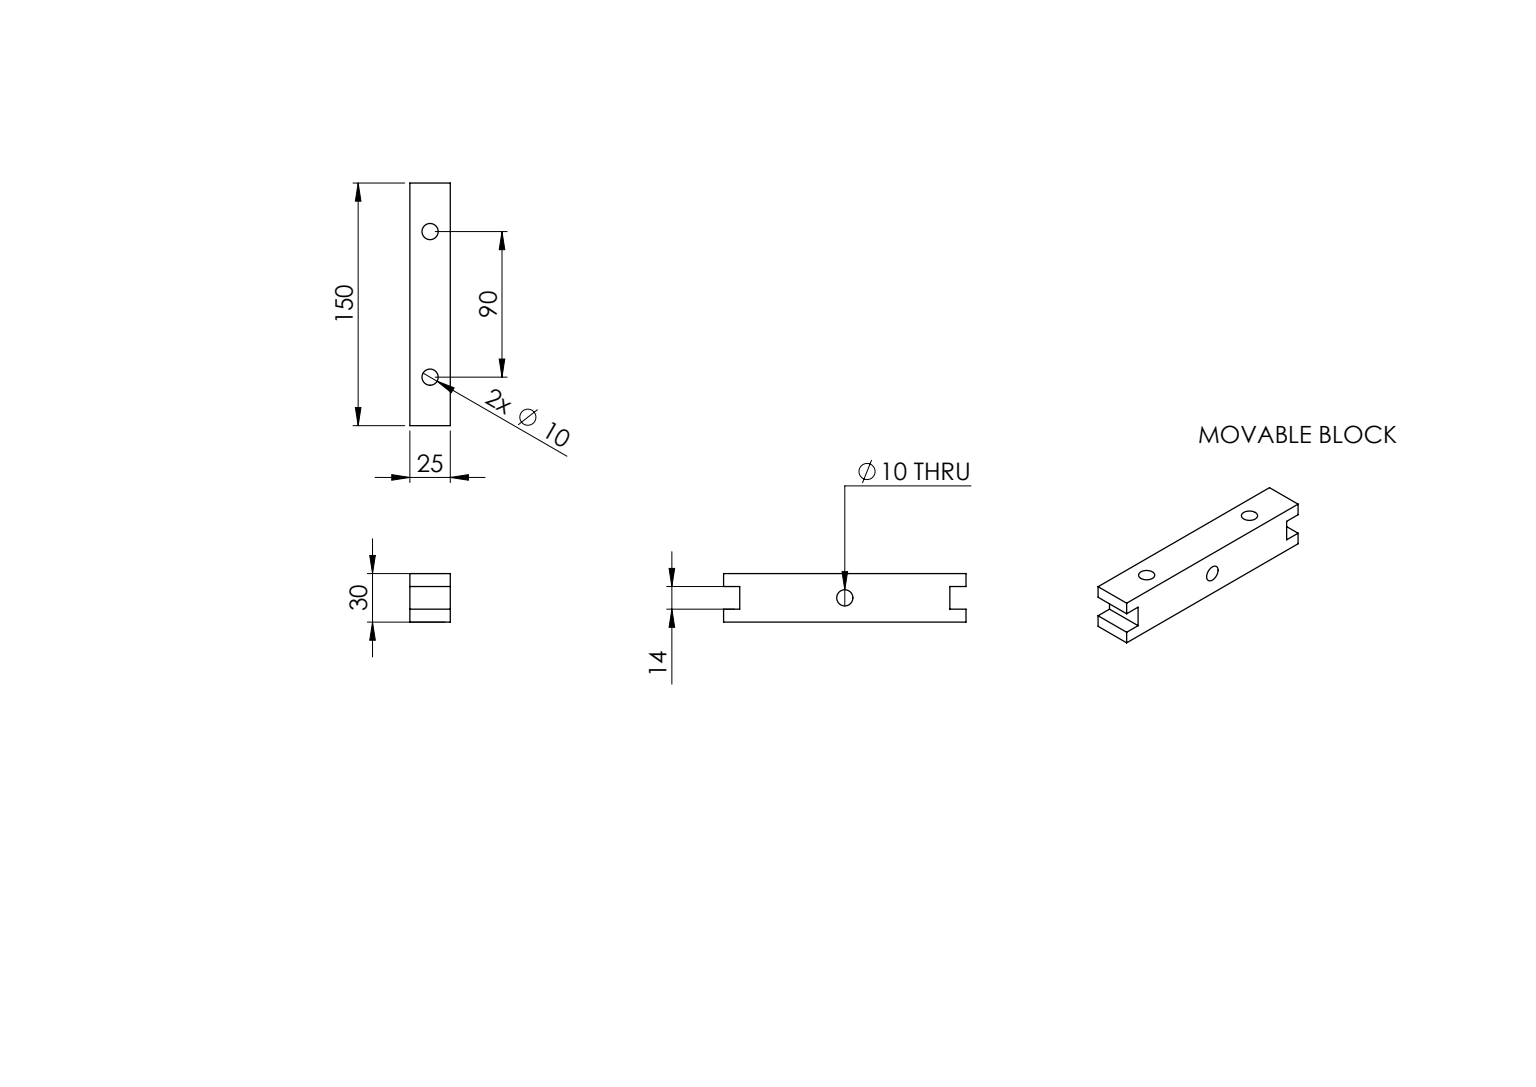
ISO-10303-21;
HEADER;
FILE_DESCRIPTION (('STEP AP214'),
    '1' );
FILE_NAME ('movable block.step',
    '2026-10-27T14:18:53',
    ( '' ),
    ( '' ),
    'SwSTEP 2.0',
    'SolidWorks 2026',
    '' );
FILE_SCHEMA (( 'AUTOMOTIVE_DESIGN' ));
ENDSEC;

DATA;
#18=ORIENTED_EDGE ( 'NONE', *, *, #5131, .T. ) ;
#31=CARTESIAN_POINT ( 'NONE',  ( 137.4999999999999716, -7.000000000000013323, 75.00000000000001421 ) ) ;
#57=DIRECTION ( 'NONE',  ( 0.000000000000000000, 0.000000000000000000, -1.000000000000000000 ) ) ;
#75=LINE ( 'NONE', #5584, #2218 ) ;
#80=DIRECTION ( 'NONE',  ( 0.000000000000000000, 1.000000000000000000, -0.000000000000000000 ) ) ;
#94=VERTEX_POINT ( 'NONE', #863 ) ;
#107=VERTEX_POINT ( 'NONE', #2804 ) ;
#121=DIRECTION ( 'NONE',  ( -1.000000000000000000, 0.000000000000000000, 0.000000000000000000 ) ) ;
#128=VERTEX_POINT ( 'NONE', #4177 ) ;
#133=ORIENTED_EDGE ( 'NONE', *, *, #2992, .F. ) ;
#145=LINE ( 'NONE', #3381, #4186 ) ;
#176=EDGE_CURVE ( 'NONE', #2634, #3745, #5619, .T. ) ;
#180=PLANE ( 'NONE',  #2511 ) ;
#191=CARTESIAN_POINT ( 'NONE',  ( 137.4999999999999716, 15.00000000000000000, 75.00000000000001421 ) ) ;
#195=AXIS2_PLACEMENT_3D ( 'NONE', #2672, #1764, #375 ) ;
#202=FACE_OUTER_BOUND ( 'NONE', #385, .T. ) ;
#204=PLANE ( 'NONE',  #1558 ) ;
#226=VECTOR ( 'NONE', #1143, 1000.000000000000000 ) ;
#233=EDGE_CURVE ( 'NONE', #2491, #3368, #3007, .T. ) ;
#243=CLOSED_SHELL ( 'NONE', ( #387, #4012, #859, #4445, #3072, #5289, #5765, #2717, #915, #3857, #5172, #2981, #4882, #2867, #4541, #2097, #5257, #5474, #4624, #721, #3860, #288 ) ) ;
#250=EDGE_LOOP ( 'NONE', ( #3367, #4044, #762, #2973 ) ) ;
#263=LINE ( 'NONE', #1654, #3890 ) ;
#272=MANIFOLD_SOLID_BREP ( 'Cut-Extrude2', #243 ) ;
#276=ORIENTED_EDGE ( 'NONE', *, *, #2236, .T. ) ;
#288=ADVANCED_FACE ( 'NONE', ( #4164 ), #2769, .F. ) ;
#296=DIRECTION ( 'NONE',  ( 0.000000000000000000, 0.000000000000000000, -1.000000000000000000 ) ) ;
#317=CARTESIAN_POINT ( 'NONE',  ( 137.4999999999999716, 15.00000000000000000, 65.00000000000000000 ) ) ;
#319=VECTOR ( 'NONE', #2665, 1000.000000000000000 ) ;
#336=AXIS2_PLACEMENT_3D ( 'NONE', #1876, #5603, #1027 ) ;
#339=DIRECTION ( 'NONE',  ( 1.000000000000000000, 0.000000000000000000, 0.000000000000000000 ) ) ;
#358=DIRECTION ( 'NONE',  ( 0.000000000000000000, 0.000000000000000000, -1.000000000000000000 ) ) ;
#375=DIRECTION ( 'NONE',  ( 0.000000000000000000, 0.000000000000000000, -1.000000000000000000 ) ) ;
#376=EDGE_LOOP ( 'NONE', ( #1948, #3141, #4446, #529, #3460, #5164, #2752, #3738, #499, #1793, #4023, #3829 ) ) ;
#381=CARTESIAN_POINT ( 'NONE',  ( 150.0000000000000284, 15.00000000000000000, 45.00000000000000000 ) ) ;
#385=EDGE_LOOP ( 'NONE', ( #2934, #576, #5503, #570 ) ) ;
#387=ADVANCED_FACE ( 'NONE', ( #827 ), #2284, .F. ) ;
#392=CARTESIAN_POINT ( 'NONE',  ( 137.4999999999999716, 15.00000000000000000, -75.00000000000000000 ) ) ;
#401=ORIENTED_EDGE ( 'NONE', *, *, #5953, .F. ) ;
#410=ORIENTED_EDGE ( 'NONE', *, *, #1827, .F. ) ;
#422=EDGE_LOOP ( 'NONE', ( #5932, #2408, #3611, #5800 ) ) ;
#425=CARTESIAN_POINT ( 'NONE',  ( 150.0000000000000284, 15.00000000000000000, -49.99999999999998579 ) ) ;
#437=CARTESIAN_POINT ( 'NONE',  ( 137.4999999999999716, 6.999999999999985789, 75.00000000000000000 ) ) ;
#439=EDGE_CURVE ( 'NONE', #128, #2057, #2951, .T. ) ;
#455=FACE_OUTER_BOUND ( 'NONE', #872, .T. ) ;
#467=VERTEX_POINT ( 'NONE', #1515 ) ;
#471=DIRECTION ( 'NONE',  ( 0.000000000000000000, 0.000000000000000000, -1.000000000000000000 ) ) ;
#499=ORIENTED_EDGE ( 'NONE', *, *, #2236, .F. ) ;
#527=DIRECTION ( 'NONE',  ( 0.000000000000000000, 0.000000000000000000, 1.000000000000000000 ) ) ;
#529=ORIENTED_EDGE ( 'NONE', *, *, #5643, .T. ) ;
#541=DIRECTION ( 'NONE',  ( 0.000000000000000000, 0.000000000000000000, 1.000000000000000000 ) ) ;
#549=DIRECTION ( 'NONE',  ( -1.000000000000000000, -0.000000000000000000, -0.000000000000000000 ) ) ;
#559=DIRECTION ( 'NONE',  ( 0.000000000000000000, 1.000000000000000000, 0.000000000000000000 ) ) ;
#562=EDGE_CURVE ( 'NONE', #4905, #467, #1144, .T. ) ;
#567=EDGE_CURVE ( 'NONE', #1705, #3162, #5290, .T. ) ;
#570=ORIENTED_EDGE ( 'NONE', *, *, #1866, .T. ) ;
#576=ORIENTED_EDGE ( 'NONE', *, *, #439, .T. ) ;
#578=EDGE_CURVE ( 'NONE', #1123, #2345, #5796, .T. ) ;
#586=ORIENTED_EDGE ( 'NONE', *, *, #4414, .F. ) ;
#595=ORIENTED_EDGE ( 'NONE', *, *, #233, .F. ) ;
#604=VECTOR ( 'NONE', #4156, 1000.000000000000000 ) ;
#605=VERTEX_POINT ( 'NONE', #5349 ) ;
#609=DIRECTION ( 'NONE',  ( 1.000000000000000000, -0.000000000000000000, 0.000000000000000000 ) ) ;
#622=ORIENTED_EDGE ( 'NONE', *, *, #578, .T. ) ;
#628=DIRECTION ( 'NONE',  ( -0.000000000000000000, -1.000000000000000000, -0.000000000000000000 ) ) ;
#629=DIRECTION ( 'NONE',  ( -0.000000000000000000, -1.000000000000000000, -0.000000000000000000 ) ) ;
#630=FACE_OUTER_BOUND ( 'NONE', #4465, .T. ) ;
#660=CARTESIAN_POINT ( 'NONE',  ( 150.0000000000000284, 15.00000000000000000, -45.00000000000000000 ) ) ;
#667=DIRECTION ( 'NONE',  ( 1.000000000000000000, 0.000000000000000000, 0.000000000000000000 ) ) ;
#674=VERTEX_POINT ( 'NONE', #3042 ) ;
#677=EDGE_CURVE ( 'NONE', #3503, #2491, #2020, .T. ) ;
#685=ORIENTED_EDGE ( 'NONE', *, *, #934, .F. ) ;
#689=VECTOR ( 'NONE', #5205, 1000.000000000000000 ) ;
#706=CARTESIAN_POINT ( 'NONE',  ( 20.85786437626904899, 0.000000000000000000, -5.000000000000000000 ) ) ;
#712=CARTESIAN_POINT ( 'NONE',  ( 137.4999999999999716, 15.00000000000000000, -75.00000000000000000 ) ) ;
#721=ADVANCED_FACE ( 'NONE', ( #2279 ), #5554, .F. ) ;
#725=DIRECTION ( 'NONE',  ( 0.000000000000000000, -1.000000000000000000, 0.000000000000000000 ) ) ;
#731=ORIENTED_EDGE ( 'NONE', *, *, #3681, .T. ) ;
#748=DIRECTION ( 'NONE',  ( 0.000000000000000000, 0.000000000000000000, -1.000000000000000000 ) ) ;
#756=ORIENTED_EDGE ( 'NONE', *, *, #1523, .T. ) ;
#762=ORIENTED_EDGE ( 'NONE', *, *, #2902, .T. ) ;
#776=DIRECTION ( 'NONE',  ( 0.000000000000000000, 1.000000000000000000, 0.000000000000000000 ) ) ;
#784=CIRCLE ( 'NONE', #2623, 4.999999999999990230 ) ;
#803=LINE ( 'NONE', #4483, #970 ) ;
#812=ORIENTED_EDGE ( 'NONE', *, *, #1765, .T. ) ;
#814=LINE ( 'NONE', #392, #319 ) ;
#816=ORIENTED_EDGE ( 'NONE', *, *, #562, .F. ) ;
#821=CARTESIAN_POINT ( 'NONE',  ( 150.0000000000000284, 15.00000000000000000, 45.00000000000000000 ) ) ;
#822=DIRECTION ( 'NONE',  ( -0.000000000000000000, -1.000000000000000000, 0.000000000000000000 ) ) ;
#827=FACE_OUTER_BOUND ( 'NONE', #1704, .T. ) ;
#849=LINE ( 'NONE', #1272, #3893 ) ;
#859=ADVANCED_FACE ( 'NONE', ( #3753 ), #1050, .F. ) ;
#863=CARTESIAN_POINT ( 'NONE',  ( 162.5000000000000000, -15.00000000000000000, 75.00000000000001421 ) ) ;
#872=EDGE_LOOP ( 'NONE', ( #4611, #1557, #18, #812 ) ) ;
#882=AXIS2_PLACEMENT_3D ( 'NONE', #928, #4615, #5515 ) ;
#893=AXIS2_PLACEMENT_3D ( 'NONE', #5598, #1393, #3728 ) ;
#896=ORIENTED_EDGE ( 'NONE', *, *, #439, .F. ) ;
#902=PLANE ( 'NONE',  #3882 ) ;
#904=CARTESIAN_POINT ( 'NONE',  ( 162.4999999999999716, 7.000000000000013323, -65.00000000000000000 ) ) ;
#915=ADVANCED_FACE ( 'NONE', ( #1931, #4768 ), #4797, .F. ) ;
#916=CARTESIAN_POINT ( 'NONE',  ( 20.85786437626904899, 0.000000000000000000, 0.000000000000000000 ) ) ;
#928=CARTESIAN_POINT ( 'NONE',  ( 24.99999999999998224, 6.999999999999985789, 75.00000000000000000 ) ) ;
#933=DIRECTION ( 'NONE',  ( 1.000000000000000000, 0.000000000000000000, -0.000000000000000000 ) ) ;
#934=EDGE_CURVE ( 'NONE', #3290, #107, #1539, .T. ) ;
#948=ORIENTED_EDGE ( 'NONE', *, *, #2872, .F. ) ;
#960=PLANE ( 'NONE',  #893 ) ;
#962=ORIENTED_EDGE ( 'NONE', *, *, #2793, .T. ) ;
#963=VECTOR ( 'NONE', #121, 1000.000000000000000 ) ;
#964=CARTESIAN_POINT ( 'NONE',  ( 137.4999999999999716, 15.00000000000000000, 75.00000000000001421 ) ) ;
#966=ORIENTED_EDGE ( 'NONE', *, *, #4593, .T. ) ;
#970=VECTOR ( 'NONE', #1314, 1000.000000000000000 ) ;
#988=CARTESIAN_POINT ( 'NONE',  ( 162.5000000000000000, -15.00000000000000000, 75.00000000000001421 ) ) ;
#989=( GEOMETRIC_REPRESENTATION_CONTEXT ( 3 ) GLOBAL_UNCERTAINTY_ASSIGNED_CONTEXT ( ( #3370 ) ) GLOBAL_UNIT_ASSIGNED_CONTEXT ( ( #3076, #3468, #4966 ) ) REPRESENTATION_CONTEXT ( 'NONE', 'WORKASPACE' ) );
#1003=ORIENTED_EDGE ( 'NONE', *, *, #1751, .F. ) ;
#1027=DIRECTION ( 'NONE',  ( 0.000000000000000000, 0.000000000000000000, -1.000000000000000000 ) ) ;
#1045=DIRECTION ( 'NONE',  ( 0.000000000000000000, 0.000000000000000000, -1.000000000000000000 ) ) ;
#1050=CYLINDRICAL_SURFACE ( 'NONE', #336, 4.999999999999990230 ) ;
#1052=VECTOR ( 'NONE', #5862, 1000.000000000000000 ) ;
#1070=FACE_OUTER_BOUND ( 'NONE', #1401, .T. ) ;
#1100=CARTESIAN_POINT ( 'NONE',  ( 24.99999999999998224, -6.999999999999985789, -75.00000000000000000 ) ) ;
#1102=DIRECTION ( 'NONE',  ( 0.000000000000000000, -1.000000000000000000, 0.000000000000000000 ) ) ;
#1104=EDGE_LOOP ( 'NONE', ( #1187, #2444 ) ) ;
#1123=VERTEX_POINT ( 'NONE', #2479 ) ;
#1133=DIRECTION ( 'NONE',  ( 1.000000000000000000, 4.770489558936219510E-17, 0.000000000000000000 ) ) ;
#1140=SURFACE_SIDE_STYLE ('',( #4859 ) ) ;
#1143=DIRECTION ( 'NONE',  ( 0.000000000000000000, -1.000000000000000000, 0.000000000000000000 ) ) ;
#1144=LINE ( 'NONE', #4865, #1905 ) ;
#1155=VERTEX_POINT ( 'NONE', #4897 ) ;
#1165=VECTOR ( 'NONE', #5568, 1000.000000000000000 ) ;
#1168=CARTESIAN_POINT ( 'NONE',  ( 137.4999999999999716, -6.999999999999985789, 75.00000000000001421 ) ) ;
#1187=ORIENTED_EDGE ( 'NONE', *, *, #2618, .T. ) ;
#1243=CARTESIAN_POINT ( 'NONE',  ( 162.5000000000000000, 15.00000000000000000, 65.00000000000000000 ) ) ;
#1272=CARTESIAN_POINT ( 'NONE',  ( 24.99999999999998224, 6.999999999999985789, 75.00000000000000000 ) ) ;
#1283=EDGE_LOOP ( 'NONE', ( #2205, #3350 ) ) ;
#1288=DIRECTION ( 'NONE',  ( 0.000000000000000000, -1.000000000000000000, 0.000000000000000000 ) ) ;
#1290=DIRECTION ( 'NONE',  ( 1.000000000000000000, 0.000000000000000000, 0.000000000000000000 ) ) ;
#1304=LINE ( 'NONE', #4061, #2536 ) ;
#1314=DIRECTION ( 'NONE',  ( 0.000000000000000000, 1.000000000000000000, 0.000000000000000000 ) ) ;
#1331=DIRECTION ( 'NONE',  ( 0.000000000000000000, 0.000000000000000000, -1.000000000000000000 ) ) ;
#1350=LINE ( 'NONE', #425, #3589 ) ;
#1354=ORIENTED_EDGE ( 'NONE', *, *, #3614, .F. ) ;
#1357=VECTOR ( 'NONE', #5280, 1000.000000000000000 ) ;
#1382=LINE ( 'NONE', #1914, #4159 ) ;
#1387=PLANE ( 'NONE',  #882 ) ;
#1393=DIRECTION ( 'NONE',  ( 4.770489558936220126E-17, -1.000000000000000000, 0.000000000000000000 ) ) ;
#1401=EDGE_LOOP ( 'NONE', ( #5118, #133, #685, #2620 ) ) ;
#1435=LINE ( 'NONE', #988, #1937 ) ;
#1441=DIRECTION ( 'NONE',  ( -1.000000000000000000, 0.000000000000000000, 0.000000000000000000 ) ) ;
#1443=VECTOR ( 'NONE', #2926, 1000.000000000000000 ) ;
#1451=EDGE_CURVE ( 'NONE', #3980, #5855, #3167, .T. ) ;
#1454=CARTESIAN_POINT ( 'NONE',  ( 150.0000000000000284, 0.000000000000000000, 40.00000000000000711 ) ) ;
#1467=ORIENTED_EDGE ( 'NONE', *, *, #176, .F. ) ;
#1477=DIRECTION ( 'NONE',  ( 1.000000000000000000, 0.000000000000000000, 0.000000000000000000 ) ) ;
#1490=EDGE_CURVE ( 'NONE', #2057, #2341, #3386, .T. ) ;
#1507=DIRECTION ( 'NONE',  ( 0.000000000000000000, -1.000000000000000000, 0.000000000000000000 ) ) ;
#1515=CARTESIAN_POINT ( 'NONE',  ( 162.4999999999999716, -6.999999999999985789, -65.00000000000000000 ) ) ;
#1523=EDGE_CURVE ( 'NONE', #1679, #4905, #2497, .T. ) ;
#1528=DIRECTION ( 'NONE',  ( 0.000000000000000000, -1.000000000000000000, 0.000000000000000000 ) ) ;
#1539=LINE ( 'NONE', #1964, #2554 ) ;
#1550=CIRCLE ( 'NONE', #5524, 4.999999999999990230 ) ;
#1551=DIRECTION ( 'NONE',  ( 0.000000000000000000, 0.000000000000000000, -1.000000000000000000 ) ) ;
#1557=ORIENTED_EDGE ( 'NONE', *, *, #1523, .F. ) ;
#1558=AXIS2_PLACEMENT_3D ( 'NONE', #2443, #1528, #4423 ) ;
#1561=CARTESIAN_POINT ( 'NONE',  ( 0.000000000000000000, 15.00000000000000000, 0.000000000000000000 ) ) ;
#1574=DIRECTION ( 'NONE',  ( 1.000000000000000000, -4.770489558936219510E-17, 0.000000000000000000 ) ) ;
#1598=CARTESIAN_POINT ( 'NONE',  ( 162.5000000000000000, 15.00000000000000000, 75.00000000000001421 ) ) ;
#1627=EDGE_LOOP ( 'NONE', ( #3281, #4685, #731, #4014 ) ) ;
#1646=EDGE_CURVE ( 'NONE', #2345, #1926, #4025, .T. ) ;
#1650=AXIS2_PLACEMENT_3D ( 'NONE', #5756, #3905, #748 ) ;
#1654=CARTESIAN_POINT ( 'NONE',  ( 162.5000000000000000, 15.00000000000000000, 75.00000000000001421 ) ) ;
#1666=DIRECTION ( 'NONE',  ( 0.000000000000000000, -1.000000000000000000, 0.000000000000000000 ) ) ;
#1679=VERTEX_POINT ( 'NONE', #4000 ) ;
#1687=FACE_OUTER_BOUND ( 'NONE', #5817, .T. ) ;
#1692=DIRECTION ( 'NONE',  ( 1.000000000000000000, -0.000000000000000000, 0.000000000000000000 ) ) ;
#1704=EDGE_LOOP ( 'NONE', ( #948, #3524, #962, #5311 ) ) ;
#1705=VERTEX_POINT ( 'NONE', #5935 ) ;
#1711=EDGE_LOOP ( 'NONE', ( #2373, #5638, #896, #4217 ) ) ;
#1713=ORIENTED_EDGE ( 'NONE', *, *, #4593, .F. ) ;
#1742=VECTOR ( 'NONE', #822, 1000.000000000000000 ) ;
#1746=CARTESIAN_POINT ( 'NONE',  ( 137.4999999999999716, -15.00000000000000000, 75.00000000000001421 ) ) ;
#1751=EDGE_CURVE ( 'NONE', #3368, #605, #4825, .T. ) ;
#1763=VECTOR ( 'NONE', #3641, 1000.000000000000000 ) ;
#1764=DIRECTION ( 'NONE',  ( 1.000000000000000000, -0.000000000000000000, 0.000000000000000000 ) ) ;
#1765=EDGE_CURVE ( 'NONE', #2341, #1155, #3185, .T. ) ;
#1767=AXIS2_PLACEMENT_3D ( 'NONE', #3848, #3734, #2368 ) ;
#1777=CARTESIAN_POINT ( 'NONE',  ( 137.4999999999999716, 15.00000000000000000, 75.00000000000001421 ) ) ;
#1778=ORIENTED_EDGE ( 'NONE', *, *, #5908, .F. ) ;
#1780=DIRECTION ( 'NONE',  ( 0.000000000000000000, 1.000000000000000000, -0.000000000000000000 ) ) ;
#1781=DIRECTION ( 'NONE',  ( 1.000000000000000000, 0.000000000000000000, -0.000000000000000000 ) ) ;
#1793=ORIENTED_EDGE ( 'NONE', *, *, #3169, .F. ) ;
#1796=DIRECTION ( 'NONE',  ( 0.000000000000000000, 0.000000000000000000, -1.000000000000000000 ) ) ;
#1798=ORIENTED_EDGE ( 'NONE', *, *, #3461, .T. ) ;
#1805=EDGE_CURVE ( 'NONE', #3531, #5881, #2606, .T. ) ;
#1808=VECTOR ( 'NONE', #1133, 1000.000000000000000 ) ;
#1815=VECTOR ( 'NONE', #2977, 1000.000000000000000 ) ;
#1819=EDGE_CURVE ( 'NONE', #467, #3160, #3328, .T. ) ;
#1820=VERTEX_POINT ( 'NONE', #2294 ) ;
#1827=EDGE_CURVE ( 'NONE', #2491, #3503, #4742, .T. ) ;
#1852=AXIS2_PLACEMENT_3D ( 'NONE', #381, #1288, #4910 ) ;
#1858=AXIS2_PLACEMENT_3D ( 'NONE', #2816, #541, #933 ) ;
#1865=DIRECTION ( 'NONE',  ( -0.000000000000000000, -1.000000000000000000, -0.000000000000000000 ) ) ;
#1866=EDGE_CURVE ( 'NONE', #2395, #4390, #1382, .T. ) ;
#1876=CARTESIAN_POINT ( 'NONE',  ( 150.0000000000000284, 15.00000000000000000, -45.00000000000000000 ) ) ;
#1882=ADVANCED_BREP_SHAPE_REPRESENTATION ( '', ( #272, #5080 ), #5457 ) ;
#1905=VECTOR ( 'NONE', #4504, 1000.000000000000000 ) ;
#1914=CARTESIAN_POINT ( 'NONE',  ( 137.4999999999999716, 15.00000000000000000, 75.00000000000001421 ) ) ;
#1924=DIRECTION ( 'NONE',  ( 0.000000000000000000, 0.000000000000000000, -1.000000000000000000 ) ) ;
#1925=EDGE_CURVE ( 'NONE', #2057, #2395, #4212, .T. ) ;
#1926=VERTEX_POINT ( 'NONE', #2352 ) ;
#1931=FACE_BOUND ( 'NONE', #1104, .T. ) ;
#1937=VECTOR ( 'NONE', #1951, 1000.000000000000000 ) ;
#1947=CARTESIAN_POINT ( 'NONE',  ( 150.0000000000000284, 15.00000000000000000, -45.00000000000000000 ) ) ;
#1948=ORIENTED_EDGE ( 'NONE', *, *, #5131, .F. ) ;
#1949=LINE ( 'NONE', #5203, #3492 ) ;
#1951=DIRECTION ( 'NONE',  ( 0.000000000000000000, 0.000000000000000000, -1.000000000000000000 ) ) ;
#1959=LINE ( 'NONE', #2848, #604 ) ;
#1964=CARTESIAN_POINT ( 'NONE',  ( 137.4999999999999716, -15.00000000000000000, 75.00000000000001421 ) ) ;
#1973=EDGE_CURVE ( 'NONE', #4267, #107, #5683, .T. ) ;
#2009=FACE_BOUND ( 'NONE', #2470, .T. ) ;
#2018=AXIS2_PLACEMENT_3D ( 'NONE', #1100, #4356, #3146 ) ;
#2020=CIRCLE ( 'NONE', #2212, 4.999999999999990230 ) ;
#2039=EDGE_LOOP ( 'NONE', ( #3911, #4544, #5055, #4116 ) ) ;
#2045=VERTEX_POINT ( 'NONE', #2957 ) ;
#2057=VERTEX_POINT ( 'NONE', #712 ) ;
#2097=ADVANCED_FACE ( 'NONE', ( #5267 ), #4748, .T. ) ;
#2115=EDGE_LOOP ( 'NONE', ( #586, #5648, #3626, #4710, #3081, #5244, #5587, #5254, #3632, #4766, #4070, #816 ) ) ;
#2129=EDGE_CURVE ( 'NONE', #4498, #94, #5409, .T. ) ;
#2153=AXIS2_PLACEMENT_3D ( 'NONE', #916, #5500, #1796 ) ;
#2158=MECHANICAL_DESIGN_GEOMETRIC_PRESENTATION_REPRESENTATION('',(#4298),#3326);
#2191=VECTOR ( 'NONE', #628, 1000.000000000000000 ) ;
#2194=FACE_OUTER_BOUND ( 'NONE', #2313, .T. ) ;
#2205=ORIENTED_EDGE ( 'NONE', *, *, #1451, .F. ) ;
#2212=AXIS2_PLACEMENT_3D ( 'NONE', #3528, #4929, #5857 ) ;
#2213=CARTESIAN_POINT ( 'NONE',  ( 150.0000000000000284, 0.000000000000000000, 45.00000000000000000 ) ) ;
#2218=VECTOR ( 'NONE', #3284, 1000.000000000000000 ) ;
#2222=DIRECTION ( 'NONE',  ( 0.000000000000000000, 0.000000000000000000, -1.000000000000000000 ) ) ;
#2233=CARTESIAN_POINT ( 'NONE',  ( 24.99999999999998224, -7.000000000000006217, 65.00000000000000000 ) ) ;
#2234=PRODUCT ( 'movable block', 'movable block', '', ( #3928 ) ) ;
#2236=EDGE_CURVE ( 'NONE', #2685, #5415, #75, .T. ) ;
#2241=ORIENTED_EDGE ( 'NONE', *, *, #4277, .T. ) ;
#2244=CARTESIAN_POINT ( 'NONE',  ( 162.5000000000000000, 15.00000000000000000, 75.00000000000001421 ) ) ;
#2279=FACE_OUTER_BOUND ( 'NONE', #5448, .T. ) ;
#2282=EDGE_LOOP ( 'NONE', ( #1467, #2674, #3212, #4607 ) ) ;
#2284=CYLINDRICAL_SURFACE ( 'NONE', #4124, 5.000000000000000000 ) ;
#2294=CARTESIAN_POINT ( 'NONE',  ( 137.4999999999999716, -6.999999999999985789, -75.00000000000000000 ) ) ;
#2295=CARTESIAN_POINT ( 'NONE',  ( 24.99999999999998224, -7.000000000000006217, 75.00000000000000000 ) ) ;
#2310=AXIS2_PLACEMENT_3D ( 'NONE', #4942, #776, #527 ) ;
#2313=EDGE_LOOP ( 'NONE', ( #3715, #966, #4508, #3808 ) ) ;
#2336=CARTESIAN_POINT ( 'NONE',  ( 150.0000000000000284, 15.00000000000000000, 49.99999999999998579 ) ) ;
#2337=AXIS2_PLACEMENT_3D ( 'NONE', #3473, #559, #5656 ) ;
#2341=VERTEX_POINT ( 'NONE', #4141 ) ;
#2345=VERTEX_POINT ( 'NONE', #5703 ) ;
#2352=CARTESIAN_POINT ( 'NONE',  ( 162.4999999999999716, 6.999999999999985789, 75.00000000000000000 ) ) ;
#2354=PLANE ( 'NONE',  #3313 ) ;
#2368=DIRECTION ( 'NONE',  ( 0.000000000000000000, 0.000000000000000000, -1.000000000000000000 ) ) ;
#2373=ORIENTED_EDGE ( 'NONE', *, *, #1765, .F. ) ;
#2379=CARTESIAN_POINT ( 'NONE',  ( 137.4999999999999716, -6.999999999999985789, -65.00000000000000000 ) ) ;
#2395=VERTEX_POINT ( 'NONE', #191 ) ;
#2408=ORIENTED_EDGE ( 'NONE', *, *, #4800, .F. ) ;
#2418=EDGE_CURVE ( 'NONE', #467, #5410, #3465, .T. ) ;
#2442=CARTESIAN_POINT ( 'NONE',  ( 162.5000000000000000, 6.123233995736766282E-16, 5.000000000000000000 ) ) ;
#2443=CARTESIAN_POINT ( 'NONE',  ( 0.000000000000000000, -15.00000000000000000, 0.000000000000000000 ) ) ;
#2444=ORIENTED_EDGE ( 'NONE', *, *, #2872, .T. ) ;
#2450=CARTESIAN_POINT ( 'NONE',  ( 150.0000000000000284, 15.00000000000000000, 49.99999999999998579 ) ) ;
#2459=CARTESIAN_POINT ( 'NONE',  ( 24.99999999999998224, 6.999999999999985789, 65.00000000000000000 ) ) ;
#2470=EDGE_LOOP ( 'NONE', ( #5525, #410 ) ) ;
#2479=CARTESIAN_POINT ( 'NONE',  ( 162.4999999999999716, -7.000000000000013323, 65.00000000000000000 ) ) ;
#2486=ORIENTED_EDGE ( 'NONE', *, *, #2522, .T. ) ;
#2491=VERTEX_POINT ( 'NONE', #5406 ) ;
#2493=PLANE ( 'NONE',  #2337 ) ;
#2496=EDGE_CURVE ( 'NONE', #5415, #674, #5023, .T. ) ;
#2497=LINE ( 'NONE', #2966, #1808 ) ;
#2506=SHAPE_REPRESENTATION_RELATIONSHIP ( 'NONE' , 'NONE' ,  #5882, #1882 ) ;
#2511=AXIS2_PLACEMENT_3D ( 'NONE', #4402, #5849, #4852 ) ;
#2522=EDGE_CURVE ( 'NONE', #5881, #3531, #1550, .T. ) ;
#2536=VECTOR ( 'NONE', #3227, 1000.000000000000000 ) ;
#2546=( NAMED_UNIT ( * ) SI_UNIT ( $, .STERADIAN. ) SOLID_ANGLE_UNIT ( ) );
#2554=VECTOR ( 'NONE', #4314, 1000.000000000000000 ) ;
#2579=DIRECTION ( 'NONE',  ( 1.000000000000000000, -0.000000000000000000, -0.000000000000000000 ) ) ;
#2580=AXIS2_PLACEMENT_3D ( 'NONE', #2786, #4641, #3477 ) ;
#2588=EDGE_LOOP ( 'NONE', ( #5585, #1354, #4536, #4616 ) ) ;
#2606=CIRCLE ( 'NONE', #2310, 4.999999999999990230 ) ;
#2618=EDGE_CURVE ( 'NONE', #1705, #2634, #4754, .T. ) ;
#2619=CARTESIAN_POINT ( 'NONE',  ( 150.0000000000000284, 15.00000000000000000, 40.00000000000000711 ) ) ;
#2620=ORIENTED_EDGE ( 'NONE', *, *, #3681, .F. ) ;
#2623=AXIS2_PLACEMENT_3D ( 'NONE', #2838, #5566, #4668 ) ;
#2634=VERTEX_POINT ( 'NONE', #4066 ) ;
#2639=STYLED_ITEM('',(#5999),#272);
#2653=APPLICATION_CONTEXT ( 'automotive_design' ) ;
#2664=DIRECTION ( 'NONE',  ( -1.000000000000000000, 4.770489558936220126E-17, 0.000000000000000000 ) ) ;
#2665=DIRECTION ( 'NONE',  ( -0.000000000000000000, -1.000000000000000000, -0.000000000000000000 ) ) ;
#2672=CARTESIAN_POINT ( 'NONE',  ( 137.4999999999999716, 0.000000000000000000, 0.000000000000000000 ) ) ;
#2674=ORIENTED_EDGE ( 'NONE', *, *, #2618, .F. ) ;
#2675=CARTESIAN_POINT ( 'NONE',  ( 20.85786437626904899, 0.000000000000000000, 0.000000000000000000 ) ) ;
#2683=PLANE ( 'NONE',  #3226 ) ;
#2685=VERTEX_POINT ( 'NONE', #437 ) ;
#2689=PLANE ( 'NONE',  #5819 ) ;
#2700=VECTOR ( 'NONE', #5392, 1000.000000000000000 ) ;
#2706=DIRECTION ( 'NONE',  ( 1.000000000000000000, -0.000000000000000000, -0.000000000000000000 ) ) ;
#2717=ADVANCED_FACE ( 'NONE', ( #3390, #4134 ), #5597, .F. ) ;
#2719=EDGE_CURVE ( 'NONE', #5410, #1820, #5160, .T. ) ;
#2752=ORIENTED_EDGE ( 'NONE', *, *, #4959, .F. ) ;
#2769=CYLINDRICAL_SURFACE ( 'NONE', #2153, 5.000000000000000000 ) ;
#2786=CARTESIAN_POINT ( 'NONE',  ( 150.0000000000000284, 15.00000000000000000, 45.00000000000000000 ) ) ;
#2793=EDGE_CURVE ( 'NONE', #3745, #3162, #3870, .T. ) ;
#2804=CARTESIAN_POINT ( 'NONE',  ( 137.4999999999999716, -15.00000000000000000, 75.00000000000001421 ) ) ;
#2810=LINE ( 'NONE', #31, #1165 ) ;
#2816=CARTESIAN_POINT ( 'NONE',  ( 137.4999999999999716, 15.00000000000000000, -75.00000000000000000 ) ) ;
#2817=AXIS2_PLACEMENT_3D ( 'NONE', #3424, #1666, #5282 ) ;
#2818=VECTOR ( 'NONE', #3451, 1000.000000000000000 ) ;
#2838=CARTESIAN_POINT ( 'NONE',  ( 150.0000000000000284, 15.00000000000000000, 45.00000000000000000 ) ) ;
#2842=ORIENTED_EDGE ( 'NONE', *, *, #2976, .F. ) ;
#2848=CARTESIAN_POINT ( 'NONE',  ( 162.5000000000000000, 7.000000000000013323, 75.00000000000001421 ) ) ;
#2867=ADVANCED_FACE ( 'NONE', ( #630 ), #180, .T. ) ;
#2872=EDGE_CURVE ( 'NONE', #2634, #1705, #4366, .T. ) ;
#2875=CARTESIAN_POINT ( 'NONE',  ( 162.4999999999999716, -7.000000000000013323, 75.00000000000000000 ) ) ;
#2882=VECTOR ( 'NONE', #2579, 1000.000000000000000 ) ;
#2902=EDGE_CURVE ( 'NONE', #1820, #3160, #5307, .T. ) ;
#2922=AXIS2_PLACEMENT_3D ( 'NONE', #3955, #4912, #1290 ) ;
#2924=AXIS2_PLACEMENT_3D ( 'NONE', #1561, #1102, #5779 ) ;
#2926=DIRECTION ( 'NONE',  ( 1.000000000000000000, -0.000000000000000000, -0.000000000000000000 ) ) ;
#2934=ORIENTED_EDGE ( 'NONE', *, *, #3915, .T. ) ;
#2951=LINE ( 'NONE', #3283, #3925 ) ;
#2957=CARTESIAN_POINT ( 'NONE',  ( 162.5000000000000000, -15.00000000000000000, -75.00000000000000000 ) ) ;
#2961=FACE_OUTER_BOUND ( 'NONE', #5295, .T. ) ;
#2966=CARTESIAN_POINT ( 'NONE',  ( 24.99999999999998224, 7.000000000000006217, -65.00000000000000000 ) ) ;
#2970=CYLINDRICAL_SURFACE ( 'NONE', #5350, 4.999999999999990230 ) ;
#2973=ORIENTED_EDGE ( 'NONE', *, *, #1819, .F. ) ;
#2976=EDGE_CURVE ( 'NONE', #3503, #605, #1350, .T. ) ;
#2977=DIRECTION ( 'NONE',  ( 0.000000000000000000, 1.000000000000000000, -0.000000000000000000 ) ) ;
#2981=ADVANCED_FACE ( 'NONE', ( #5936 ), #902, .T. ) ;
#2992=EDGE_CURVE ( 'NONE', #107, #94, #5898, .T. ) ;
#3007=LINE ( 'NONE', #3436, #226 ) ;
#3042=CARTESIAN_POINT ( 'NONE',  ( 137.4999999999999716, -7.000000000000011546, 65.00000000000000000 ) ) ;
#3047=DIRECTION ( 'NONE',  ( 0.000000000000000000, 0.000000000000000000, 1.000000000000000000 ) ) ;
#3072=ADVANCED_FACE ( 'NONE', ( #3086 ), #2689, .F. ) ;
#3076=( LENGTH_UNIT ( ) NAMED_UNIT ( * ) SI_UNIT ( .MILLI., .METRE. ) );
#3081=ORIENTED_EDGE ( 'NONE', *, *, #1646, .F. ) ;
#3086=FACE_OUTER_BOUND ( 'NONE', #1627, .T. ) ;
#3094=EDGE_CURVE ( 'NONE', #5855, #3980, #784, .T. ) ;
#3098=ORIENTED_EDGE ( 'NONE', *, *, #1827, .T. ) ;
#3107=PRODUCT_DEFINITION_SHAPE ( 'NONE', 'NONE',  #3939 ) ;
#3123=DIRECTION ( 'NONE',  ( 1.000000000000000000, -4.770489558936219510E-17, 0.000000000000000000 ) ) ;
#3141=ORIENTED_EDGE ( 'NONE', *, *, #3461, .F. ) ;
#3146=DIRECTION ( 'NONE',  ( 0.000000000000000000, 0.000000000000000000, 1.000000000000000000 ) ) ;
#3148=CARTESIAN_POINT ( 'NONE',  ( 150.0000000000000284, 0.000000000000000000, 49.99999999999998579 ) ) ;
#3150=ORIENTED_EDGE ( 'NONE', *, *, #3094, .T. ) ;
#3160=VERTEX_POINT ( 'NONE', #2379 ) ;
#3162=VERTEX_POINT ( 'NONE', #5623 ) ;
#3167=CIRCLE ( 'NONE', #2580, 4.999999999999990230 ) ;
#3169=EDGE_CURVE ( 'NONE', #2395, #2685, #1949, .T. ) ;
#3185=LINE ( 'NONE', #5484, #5487 ) ;
#3199=EDGE_LOOP ( 'NONE', ( #5887, #3334 ) ) ;
#3209=EDGE_LOOP ( 'NONE', ( #5087, #5799 ) ) ;
#3212=ORIENTED_EDGE ( 'NONE', *, *, #567, .T. ) ;
#3226=AXIS2_PLACEMENT_3D ( 'NONE', #1777, #358, #5449 ) ;
#3227=DIRECTION ( 'NONE',  ( 0.000000000000000000, 0.000000000000000000, -1.000000000000000000 ) ) ;
#3244=CARTESIAN_POINT ( 'NONE',  ( 137.4999999999999716, 15.00000000000000000, 75.00000000000001421 ) ) ;
#3255=ORIENTED_EDGE ( 'NONE', *, *, #1819, .T. ) ;
#3268=CARTESIAN_POINT ( 'NONE',  ( 24.99999999999998224, -6.999999999999985789, -65.00000000000000000 ) ) ;
#3281=ORIENTED_EDGE ( 'NONE', *, *, #2719, .F. ) ;
#3283=CARTESIAN_POINT ( 'NONE',  ( 137.4999999999999716, 15.00000000000000000, -75.00000000000000000 ) ) ;
#3284=DIRECTION ( 'NONE',  ( 0.000000000000000000, 0.000000000000000000, -1.000000000000000000 ) ) ;
#3290=VERTEX_POINT ( 'NONE', #3445 ) ;
#3294=DIRECTION ( 'NONE',  ( -1.000000000000000000, 0.000000000000000000, -0.000000000000000000 ) ) ;
#3313=AXIS2_PLACEMENT_3D ( 'NONE', #4215, #57, #3294 ) ;
#3318=EDGE_CURVE ( 'NONE', #5410, #2045, #3923, .T. ) ;
#3325=CARTESIAN_POINT ( 'NONE',  ( 20.85786437626904899, 6.123233995736766282E-16, 5.000000000000000000 ) ) ;
#3326=( GEOMETRIC_REPRESENTATION_CONTEXT ( 3 ) GLOBAL_UNCERTAINTY_ASSIGNED_CONTEXT ( ( #3784 ) ) GLOBAL_UNIT_ASSIGNED_CONTEXT ( ( #4436, #3937, #2546 ) ) REPRESENTATION_CONTEXT ( 'NONE', 'WORKASPACE' ) );
#3328=LINE ( 'NONE', #3268, #3672 ) ;
#3334=ORIENTED_EDGE ( 'NONE', *, *, #2793, .F. ) ;
#3338=FACE_OUTER_BOUND ( 'NONE', #1711, .T. ) ;
#3350=ORIENTED_EDGE ( 'NONE', *, *, #3094, .F. ) ;
#3367=ORIENTED_EDGE ( 'NONE', *, *, #2418, .T. ) ;
#3368=VERTEX_POINT ( 'NONE', #4449 ) ;
#3370=UNCERTAINTY_MEASURE_WITH_UNIT (LENGTH_MEASURE( 1.000000000000000082E-05 ), #3076, 'distance_accuracy_value', 'NONE');
#3381=CARTESIAN_POINT ( 'NONE',  ( 137.4999999999999716, 7.000000000000011546, 75.00000000000001421 ) ) ;
#3386=LINE ( 'NONE', #3958, #2191 ) ;
#3390=FACE_BOUND ( 'NONE', #3199, .T. ) ;
#3392=PLANE ( 'NONE',  #2817 ) ;
#3403=VECTOR ( 'NONE', #629, 1000.000000000000000 ) ;
#3412=AXIS2_PLACEMENT_3D ( 'NONE', #4250, #1477, #1924 ) ;
#3421=LINE ( 'NONE', #3478, #2818 ) ;
#3423=FACE_OUTER_BOUND ( 'NONE', #3586, .T. ) ;
#3424=CARTESIAN_POINT ( 'NONE',  ( 150.0000000000000284, 0.000000000000000000, -45.00000000000000000 ) ) ;
#3431=PRESENTATION_STYLE_ASSIGNMENT (( #5729 ) ) ;
#3436=CARTESIAN_POINT ( 'NONE',  ( 150.0000000000000284, 15.00000000000000000, -40.00000000000000711 ) ) ;
#3445=CARTESIAN_POINT ( 'NONE',  ( 137.4999999999999716, -15.00000000000000000, -75.00000000000000000 ) ) ;
#3451=DIRECTION ( 'NONE',  ( -1.000000000000000000, -0.000000000000000000, -0.000000000000000000 ) ) ;
#3454=LINE ( 'NONE', #2450, #3593 ) ;
#3460=ORIENTED_EDGE ( 'NONE', *, *, #934, .T. ) ;
#3461=EDGE_CURVE ( 'NONE', #3160, #1679, #803, .T. ) ;
#3465=LINE ( 'NONE', #4291, #4464 ) ;
#3468=( NAMED_UNIT ( * ) PLANE_ANGLE_UNIT ( ) SI_UNIT ( $, .RADIAN. ) );
#3472=DIRECTION ( 'NONE',  ( -0.000000000000000000, -1.000000000000000000, -0.000000000000000000 ) ) ;
#3473=CARTESIAN_POINT ( 'NONE',  ( 150.0000000000000284, 0.000000000000000000, 45.00000000000000000 ) ) ;
#3477=DIRECTION ( 'NONE',  ( 0.000000000000000000, 0.000000000000000000, 1.000000000000000000 ) ) ;
#3478=CARTESIAN_POINT ( 'NONE',  ( 137.4999999999999716, -15.00000000000000000, -75.00000000000000000 ) ) ;
#3492=VECTOR ( 'NONE', #1865, 1000.000000000000000 ) ;
#3495=ORIENTED_EDGE ( 'NONE', *, *, #2496, .T. ) ;
#3502=CARTESIAN_POINT ( 'NONE',  ( 162.5000000000000000, 15.00000000000000000, 75.00000000000001421 ) ) ;
#3503=VERTEX_POINT ( 'NONE', #5446 ) ;
#3518=CARTESIAN_POINT ( 'NONE',  ( 24.99999999999998224, -7.000000000000006217, 75.00000000000000000 ) ) ;
#3524=ORIENTED_EDGE ( 'NONE', *, *, #176, .T. ) ;
#3527=CARTESIAN_POINT ( 'NONE',  ( 0.000000000000000000, 0.000000000000000000, 0.000000000000000000 ) ) ;
#3528=CARTESIAN_POINT ( 'NONE',  ( 150.0000000000000284, 15.00000000000000000, -45.00000000000000000 ) ) ;
#3529=DIRECTION ( 'NONE',  ( 0.000000000000000000, 1.000000000000000000, 0.000000000000000000 ) ) ;
#3531=VERTEX_POINT ( 'NONE', #3148 ) ;
#3544=CARTESIAN_POINT ( 'NONE',  ( 162.5000000000000000, 6.999999999999985789, 75.00000000000001421 ) ) ;
#3570=DIRECTION ( 'NONE',  ( 0.000000000000000000, 0.000000000000000000, 1.000000000000000000 ) ) ;
#3586=EDGE_LOOP ( 'NONE', ( #595, #3098, #5860, #1003 ) ) ;
#3589=VECTOR ( 'NONE', #4051, 1000.000000000000000 ) ;
#3593=VECTOR ( 'NONE', #725, 1000.000000000000000 ) ;
#3611=ORIENTED_EDGE ( 'NONE', *, *, #4959, .T. ) ;
#3613=DIRECTION ( 'NONE',  ( -1.000000000000000000, -0.000000000000000000, -0.000000000000000000 ) ) ;
#3614=EDGE_CURVE ( 'NONE', #4390, #1926, #5306, .T. ) ;
#3626=ORIENTED_EDGE ( 'NONE', *, *, #3915, .F. ) ;
#3632=ORIENTED_EDGE ( 'NONE', *, *, #5032, .T. ) ;
#3641=DIRECTION ( 'NONE',  ( 0.000000000000000000, -1.000000000000000000, 0.000000000000000000 ) ) ;
#3672=VECTOR ( 'NONE', #3688, 1000.000000000000000 ) ;
#3681=EDGE_CURVE ( 'NONE', #2045, #3290, #3421, .T. ) ;
#3688=DIRECTION ( 'NONE',  ( -1.000000000000000000, 0.000000000000000000, 0.000000000000000000 ) ) ;
#3692=FACE_OUTER_BOUND ( 'NONE', #2588, .T. ) ;
#3715=ORIENTED_EDGE ( 'NONE', *, *, #1451, .T. ) ;
#3723=FACE_OUTER_BOUND ( 'NONE', #5407, .T. ) ;
#3728=DIRECTION ( 'NONE',  ( -1.000000000000000000, -4.770489558936220126E-17, 0.000000000000000000 ) ) ;
#3734=DIRECTION ( 'NONE',  ( 0.000000000000000000, 1.000000000000000000, -0.000000000000000000 ) ) ;
#3738=ORIENTED_EDGE ( 'NONE', *, *, #2496, .F. ) ;
#3745=VERTEX_POINT ( 'NONE', #2442 ) ;
#3753=FACE_OUTER_BOUND ( 'NONE', #4233, .T. ) ;
#3758=DIRECTION ( 'NONE',  ( -1.000000000000000000, -0.000000000000000000, -0.000000000000000000 ) ) ;
#3766=DIRECTION ( 'NONE',  ( 1.000000000000000000, 0.000000000000000000, 0.000000000000000000 ) ) ;
#3777=CARTESIAN_POINT ( 'NONE',  ( 162.5000000000000000, 15.00000000000000000, 75.00000000000001421 ) ) ;
#3784=UNCERTAINTY_MEASURE_WITH_UNIT (LENGTH_MEASURE( 1.000000000000000082E-05 ), #4436, 'distance_accuracy_value', 'NONE');
#3796=CIRCLE ( 'NONE', #1767, 4.999999999999990230 ) ;
#3801=EDGE_CURVE ( 'NONE', #128, #1155, #4842, .T. ) ;
#3808=ORIENTED_EDGE ( 'NONE', *, *, #4277, .F. ) ;
#3816=( LENGTH_UNIT ( ) NAMED_UNIT ( * ) SI_UNIT ( .MILLI., .METRE. ) );
#3829=ORIENTED_EDGE ( 'NONE', *, *, #1490, .T. ) ;
#3848=CARTESIAN_POINT ( 'NONE',  ( 150.0000000000000284, 0.000000000000000000, -45.00000000000000000 ) ) ;
#3857=ADVANCED_FACE ( 'NONE', ( #3924, #2009, #202 ), #3861, .F. ) ;
#3860=ADVANCED_FACE ( 'NONE', ( #2961 ), #2493, .T. ) ;
#3861=PLANE ( 'NONE',  #2924 ) ;
#3870=CIRCLE ( 'NONE', #1650, 5.000000000000000000 ) ;
#3876=FILL_AREA_STYLE ('',( #5286 ) ) ;
#3882=AXIS2_PLACEMENT_3D ( 'NONE', #2295, #5073, #2664 ) ;
#3887=APPLICATION_CONTEXT ( 'automotive_design' ) ;
#3889=ORIENTED_EDGE ( 'NONE', *, *, #233, .T. ) ;
#3890=VECTOR ( 'NONE', #2222, 1000.000000000000000 ) ;
#3892=VECTOR ( 'NONE', #549, 1000.000000000000000 ) ;
#3893=VECTOR ( 'NONE', #3613, 1000.000000000000000 ) ;
#3905=DIRECTION ( 'NONE',  ( 1.000000000000000000, 0.000000000000000000, 0.000000000000000000 ) ) ;
#3911=ORIENTED_EDGE ( 'NONE', *, *, #4621, .F. ) ;
#3915=EDGE_CURVE ( 'NONE', #4390, #128, #263, .T. ) ;
#3919=ORIENTED_EDGE ( 'NONE', *, *, #562, .T. ) ;
#3921=DIRECTION ( 'NONE',  ( -0.000000000000000000, -1.000000000000000000, -0.000000000000000000 ) ) ;
#3923=LINE ( 'NONE', #4814, #3976 ) ;
#3924=FACE_BOUND ( 'NONE', #1283, .T. ) ;
#3925=VECTOR ( 'NONE', #3758, 1000.000000000000000 ) ;
#3928=PRODUCT_CONTEXT ( 'NONE', #2653, 'mechanical' ) ;
#3931=CARTESIAN_POINT ( 'NONE',  ( 137.4999999999999716, 0.000000000000000000, 0.000000000000000000 ) ) ;
#3937=( NAMED_UNIT ( * ) PLANE_ANGLE_UNIT ( ) SI_UNIT ( $, .RADIAN. ) );
#3939=PRODUCT_DEFINITION ( 'UNKNOWN', '', #4009, #4410 ) ;
#3955=CARTESIAN_POINT ( 'NONE',  ( 0.000000000000000000, 0.000000000000000000, -65.00000000000000000 ) ) ;
#3958=CARTESIAN_POINT ( 'NONE',  ( 137.4999999999999716, 15.00000000000000000, -75.00000000000000000 ) ) ;
#3963=AXIS2_PLACEMENT_3D ( 'NONE', #1947, #80, #471 ) ;
#3976=VECTOR ( 'NONE', #3472, 1000.000000000000000 ) ;
#3980=VERTEX_POINT ( 'NONE', #2619 ) ;
#3992=FACE_OUTER_BOUND ( 'NONE', #2039, .T. ) ;
#4000=CARTESIAN_POINT ( 'NONE',  ( 137.4999999999999716, 7.000000000000011546, -65.00000000000000000 ) ) ;
#4009=PRODUCT_DEFINITION_FORMATION_WITH_SPECIFIED_SOURCE ( 'ANY', '', #2234, .NOT_KNOWN. ) ;
#4012=ADVANCED_FACE ( 'NONE', ( #2194 ), #5891, .F. ) ;
#4014=ORIENTED_EDGE ( 'NONE', *, *, #5643, .F. ) ;
#4023=ORIENTED_EDGE ( 'NONE', *, *, #1925, .F. ) ;
#4025=LINE ( 'NONE', #3544, #2700 ) ;
#4026=DIRECTION ( 'NONE',  ( 1.000000000000000000, 4.770489558936219510E-17, 0.000000000000000000 ) ) ;
#4034=CARTESIAN_POINT ( 'NONE',  ( 150.0000000000000284, 15.00000000000000000, 40.00000000000000711 ) ) ;
#4044=ORIENTED_EDGE ( 'NONE', *, *, #2719, .T. ) ;
#4051=DIRECTION ( 'NONE',  ( 0.000000000000000000, -1.000000000000000000, 0.000000000000000000 ) ) ;
#4061=CARTESIAN_POINT ( 'NONE',  ( 162.5000000000000000, -7.000000000000013323, 75.00000000000001421 ) ) ;
#4066=CARTESIAN_POINT ( 'NONE',  ( 137.4999999999999716, 6.123233995736766282E-16, 5.000000000000000000 ) ) ;
#4070=ORIENTED_EDGE ( 'NONE', *, *, #2418, .F. ) ;
#4116=ORIENTED_EDGE ( 'NONE', *, *, #2129, .F. ) ;
#4124=AXIS2_PLACEMENT_3D ( 'NONE', #2675, #2706, #4139 ) ;
#4130=LINE ( 'NONE', #4034, #1763 ) ;
#4134=FACE_OUTER_BOUND ( 'NONE', #2115, .T. ) ;
#4139=DIRECTION ( 'NONE',  ( 0.000000000000000000, 0.000000000000000000, -1.000000000000000000 ) ) ;
#4141=CARTESIAN_POINT ( 'NONE',  ( 137.4999999999999716, 7.000000000000011546, -75.00000000000000000 ) ) ;
#4156=DIRECTION ( 'NONE',  ( 0.000000000000000000, 0.000000000000000000, 1.000000000000000000 ) ) ;
#4159=VECTOR ( 'NONE', #3766, 1000.000000000000000 ) ;
#4162=AXIS2_PLACEMENT_3D ( 'NONE', #821, #5495, #1331 ) ;
#4164=FACE_OUTER_BOUND ( 'NONE', #2282, .T. ) ;
#4177=CARTESIAN_POINT ( 'NONE',  ( 162.5000000000000000, 15.00000000000000000, -75.00000000000000000 ) ) ;
#4186=VECTOR ( 'NONE', #4333, 1000.000000000000000 ) ;
#4212=LINE ( 'NONE', #3244, #5220 ) ;
#4215=CARTESIAN_POINT ( 'NONE',  ( 137.4999999999999716, 15.00000000000000000, 75.00000000000001421 ) ) ;
#4217=ORIENTED_EDGE ( 'NONE', *, *, #3801, .T. ) ;
#4233=EDGE_LOOP ( 'NONE', ( #5725, #3889, #1778, #2842 ) ) ;
#4243=AXIS2_PLACEMENT_3D ( 'NONE', #4456, #1780, #296 ) ;
#4250=CARTESIAN_POINT ( 'NONE',  ( 162.5000000000000000, 0.000000000000000000, 0.000000000000000000 ) ) ;
#4267=VERTEX_POINT ( 'NONE', #5494 ) ;
#4275=CARTESIAN_POINT ( 'NONE',  ( 24.99999999999998224, -6.999999999999985789, -75.00000000000000000 ) ) ;
#4277=EDGE_CURVE ( 'NONE', #3980, #5881, #4130, .T. ) ;
#4291=CARTESIAN_POINT ( 'NONE',  ( 162.5000000000000000, -6.999999999999985789, 75.00000000000001421 ) ) ;
#4293=EDGE_CURVE ( 'NONE', #4498, #1123, #1304, .T. ) ;
#4298=STYLED_ITEM ( 'NONE', ( #3431 ), #1882 ) ;
#4314=DIRECTION ( 'NONE',  ( -0.000000000000000000, -0.000000000000000000, 1.000000000000000000 ) ) ;
#4323=EDGE_CURVE ( 'NONE', #1926, #2685, #849, .T. ) ;
#4333=DIRECTION ( 'NONE',  ( 0.000000000000000000, 0.000000000000000000, -1.000000000000000000 ) ) ;
#4346=UNCERTAINTY_MEASURE_WITH_UNIT (LENGTH_MEASURE( 1.000000000000000082E-05 ), #3816, 'distance_accuracy_value', 'NONE');
#4356=DIRECTION ( 'NONE',  ( 0.000000000000000000, 1.000000000000000000, 0.000000000000000000 ) ) ;
#4361=ORIENTED_EDGE ( 'NONE', *, *, #1805, .F. ) ;
#4366=CIRCLE ( 'NONE', #5906, 5.000000000000000000 ) ;
#4389=CARTESIAN_POINT ( 'NONE',  ( 137.4999999999999716, 15.00000000000000000, 75.00000000000001421 ) ) ;
#4390=VERTEX_POINT ( 'NONE', #2244 ) ;
#4392=CARTESIAN_POINT ( 'NONE',  ( 162.5000000000000000, 15.00000000000000000, -75.00000000000000000 ) ) ;
#4402=CARTESIAN_POINT ( 'NONE',  ( 0.000000000000000000, 0.000000000000000000, 65.00000000000000000 ) ) ;
#4410=PRODUCT_DEFINITION_CONTEXT ( 'detailed design', #3887, 'design' ) ;
#4414=EDGE_CURVE ( 'NONE', #1155, #4905, #1959, .T. ) ;
#4423=DIRECTION ( 'NONE',  ( 0.000000000000000000, -0.000000000000000000, -1.000000000000000000 ) ) ;
#4432=EDGE_CURVE ( 'NONE', #3162, #3745, #4870, .T. ) ;
#4436=( LENGTH_UNIT ( ) NAMED_UNIT ( * ) SI_UNIT ( .MILLI., .METRE. ) );
#4445=ADVANCED_FACE ( 'NONE', ( #3338 ), #5187, .F. ) ;
#4446=ORIENTED_EDGE ( 'NONE', *, *, #2902, .F. ) ;
#4449=CARTESIAN_POINT ( 'NONE',  ( 150.0000000000000284, 0.000000000000000000, -40.00000000000000711 ) ) ;
#4456=CARTESIAN_POINT ( 'NONE',  ( 150.0000000000000284, 0.000000000000000000, -45.00000000000000000 ) ) ;
#4459=LINE ( 'NONE', #2233, #4476 ) ;
#4464=VECTOR ( 'NONE', #1551, 1000.000000000000000 ) ;
#4465=EDGE_LOOP ( 'NONE', ( #622, #5667, #3495, #5091 ) ) ;
#4476=VECTOR ( 'NONE', #3123, 1000.000000000000000 ) ;
#4483=CARTESIAN_POINT ( 'NONE',  ( 137.4999999999999716, 15.00000000000000000, -65.00000000000000000 ) ) ;
#4498=VERTEX_POINT ( 'NONE', #2875 ) ;
#4504=DIRECTION ( 'NONE',  ( 0.000000000000000000, -1.000000000000000000, 0.000000000000000000 ) ) ;
#4508=ORIENTED_EDGE ( 'NONE', *, *, #2522, .F. ) ;
#4536=ORIENTED_EDGE ( 'NONE', *, *, #1866, .F. ) ;
#4541=ADVANCED_FACE ( 'NONE', ( #455 ), #960, .T. ) ;
#4544=ORIENTED_EDGE ( 'NONE', *, *, #1973, .T. ) ;
#4565=ORIENTED_EDGE ( 'NONE', *, *, #1646, .T. ) ;
#4593=EDGE_CURVE ( 'NONE', #5855, #3531, #3454, .T. ) ;
#4607=ORIENTED_EDGE ( 'NONE', *, *, #4432, .T. ) ;
#4611=ORIENTED_EDGE ( 'NONE', *, *, #4414, .T. ) ;
#4615=DIRECTION ( 'NONE',  ( 0.000000000000000000, -1.000000000000000000, 0.000000000000000000 ) ) ;
#4616=ORIENTED_EDGE ( 'NONE', *, *, #3169, .T. ) ;
#4621=EDGE_CURVE ( 'NONE', #4267, #4498, #5758, .T. ) ;
#4624=ADVANCED_FACE ( 'NONE', ( #5340 ), #3392, .F. ) ;
#4635=DIRECTION ( 'NONE',  ( -0.000000000000000000, -0.000000000000000000, 1.000000000000000000 ) ) ;
#4641=DIRECTION ( 'NONE',  ( 0.000000000000000000, 1.000000000000000000, 0.000000000000000000 ) ) ;
#4644=( NAMED_UNIT ( * ) PLANE_ANGLE_UNIT ( ) SI_UNIT ( $, .RADIAN. ) );
#4659=ORIENTED_EDGE ( 'NONE', *, *, #1805, .T. ) ;
#4668=DIRECTION ( 'NONE',  ( 0.000000000000000000, 0.000000000000000000, 1.000000000000000000 ) ) ;
#4685=ORIENTED_EDGE ( 'NONE', *, *, #3318, .T. ) ;
#4710=ORIENTED_EDGE ( 'NONE', *, *, #3614, .T. ) ;
#4714=LINE ( 'NONE', #2459, #3892 ) ;
#4742=CIRCLE ( 'NONE', #3963, 4.999999999999990230 ) ;
#4748=PLANE ( 'NONE',  #2018 ) ;
#4754=CIRCLE ( 'NONE', #195, 5.000000000000000000 ) ;
#4766=ORIENTED_EDGE ( 'NONE', *, *, #3318, .F. ) ;
#4768=FACE_OUTER_BOUND ( 'NONE', #376, .T. ) ;
#4797=PLANE ( 'NONE',  #5649 ) ;
#4800=EDGE_CURVE ( 'NONE', #674, #1123, #4459, .T. ) ;
#4814=CARTESIAN_POINT ( 'NONE',  ( 162.5000000000000000, 15.00000000000000000, -75.00000000000000000 ) ) ;
#4822=CARTESIAN_POINT ( 'NONE',  ( 162.4999999999999716, -6.999999999999985789, -75.00000000000000000 ) ) ;
#4825=CIRCLE ( 'NONE', #4243, 4.999999999999990230 ) ;
#4831=DIRECTION ( 'NONE',  ( 0.000000000000000000, 0.000000000000000000, 1.000000000000000000 ) ) ;
#4842=LINE ( 'NONE', #4392, #689 ) ;
#4852=DIRECTION ( 'NONE',  ( 1.000000000000000000, 0.000000000000000000, -0.000000000000000000 ) ) ;
#4859=SURFACE_STYLE_FILL_AREA ( #3876 ) ;
#4865=CARTESIAN_POINT ( 'NONE',  ( 162.5000000000000000, 15.00000000000000000, -65.00000000000000000 ) ) ;
#4870=CIRCLE ( 'NONE', #3412, 5.000000000000000000 ) ;
#4882=ADVANCED_FACE ( 'NONE', ( #3723 ), #1387, .T. ) ;
#4897=CARTESIAN_POINT ( 'NONE',  ( 162.4999999999999716, 7.000000000000013323, -75.00000000000000000 ) ) ;
#4905=VERTEX_POINT ( 'NONE', #904 ) ;
#4910=DIRECTION ( 'NONE',  ( 0.000000000000000000, 0.000000000000000000, -1.000000000000000000 ) ) ;
#4912=DIRECTION ( 'NONE',  ( 0.000000000000000000, 0.000000000000000000, -1.000000000000000000 ) ) ;
#4929=DIRECTION ( 'NONE',  ( 0.000000000000000000, 1.000000000000000000, -0.000000000000000000 ) ) ;
#4942=CARTESIAN_POINT ( 'NONE',  ( 150.0000000000000284, 0.000000000000000000, 45.00000000000000000 ) ) ;
#4944=CARTESIAN_POINT ( 'NONE',  ( 137.4999999999999716, 15.00000000000000000, -75.00000000000000000 ) ) ;
#4947=VECTOR ( 'NONE', #3921, 1000.000000000000000 ) ;
#4959=EDGE_CURVE ( 'NONE', #674, #4267, #2810, .T. ) ;
#4966=( NAMED_UNIT ( * ) SI_UNIT ( $, .STERADIAN. ) SOLID_ANGLE_UNIT ( ) );
#5023=LINE ( 'NONE', #317, #1742 ) ;
#5032=EDGE_CURVE ( 'NONE', #94, #2045, #1435, .T. ) ;
#5055=ORIENTED_EDGE ( 'NONE', *, *, #2992, .T. ) ;
#5073=DIRECTION ( 'NONE',  ( 4.770489558936220126E-17, 1.000000000000000000, -0.000000000000000000 ) ) ;
#5080=AXIS2_PLACEMENT_3D ( 'NONE', #3527, #4831, #667 ) ;
#5087=ORIENTED_EDGE ( 'NONE', *, *, #5908, .T. ) ;
#5091=ORIENTED_EDGE ( 'NONE', *, *, #4800, .T. ) ;
#5118=ORIENTED_EDGE ( 'NONE', *, *, #5032, .F. ) ;
#5131=EDGE_CURVE ( 'NONE', #1679, #2341, #145, .T. ) ;
#5160=LINE ( 'NONE', #4275, #963 ) ;
#5164=ORIENTED_EDGE ( 'NONE', *, *, #1973, .F. ) ;
#5172=ADVANCED_FACE ( 'NONE', ( #1070 ), #204, .T. ) ;
#5187=PLANE ( 'NONE',  #1858 ) ;
#5203=CARTESIAN_POINT ( 'NONE',  ( 137.4999999999999716, 15.00000000000000000, 75.00000000000001421 ) ) ;
#5205=DIRECTION ( 'NONE',  ( -0.000000000000000000, -1.000000000000000000, -0.000000000000000000 ) ) ;
#5220=VECTOR ( 'NONE', #4635, 1000.000000000000000 ) ;
#5241=CARTESIAN_POINT ( 'NONE',  ( 137.4999999999999716, 6.999999999999985789, 65.00000000000000000 ) ) ;
#5244=ORIENTED_EDGE ( 'NONE', *, *, #578, .F. ) ;
#5254=ORIENTED_EDGE ( 'NONE', *, *, #2129, .T. ) ;
#5257=ADVANCED_FACE ( 'NONE', ( #1687 ), #5363, .T. ) ;
#5264=ORIENTED_EDGE ( 'NONE', *, *, #4323, .T. ) ;
#5267=FACE_OUTER_BOUND ( 'NONE', #250, .T. ) ;
#5280=DIRECTION ( 'NONE',  ( -0.000000000000000000, 0.000000000000000000, 1.000000000000000000 ) ) ;
#5282=DIRECTION ( 'NONE',  ( 0.000000000000000000, -0.000000000000000000, -1.000000000000000000 ) ) ;
#5286=FILL_AREA_STYLE_COLOUR ( '', #5939 ) ;
#5289=ADVANCED_FACE ( 'NONE', ( #3992 ), #2683, .F. ) ;
#5290=LINE ( 'NONE', #706, #2882 ) ;
#5295=EDGE_LOOP ( 'NONE', ( #2486, #4659 ) ) ;
#5306=LINE ( 'NONE', #1598, #3403 ) ;
#5307=LINE ( 'NONE', #1168, #1357 ) ;
#5311=ORIENTED_EDGE ( 'NONE', *, *, #567, .F. ) ;
#5333=SHAPE_DEFINITION_REPRESENTATION ( #3107, #5882 ) ;
#5340=FACE_OUTER_BOUND ( 'NONE', #3209, .T. ) ;
#5346=VECTOR ( 'NONE', #1574, 1000.000000000000000 ) ;
#5349=CARTESIAN_POINT ( 'NONE',  ( 150.0000000000000284, 0.000000000000000000, -49.99999999999998579 ) ) ;
#5350=AXIS2_PLACEMENT_3D ( 'NONE', #660, #1507, #1045 ) ;
#5363=PLANE ( 'NONE',  #2922 ) ;
#5392=DIRECTION ( 'NONE',  ( 0.000000000000000000, 0.000000000000000000, 1.000000000000000000 ) ) ;
#5406=CARTESIAN_POINT ( 'NONE',  ( 150.0000000000000284, 15.00000000000000000, -40.00000000000000711 ) ) ;
#5407=EDGE_LOOP ( 'NONE', ( #4565, #5264, #276, #401 ) ) ;
#5409=LINE ( 'NONE', #3502, #1052 ) ;
#5410=VERTEX_POINT ( 'NONE', #4822 ) ;
#5415=VERTEX_POINT ( 'NONE', #5241 ) ;
#5446=CARTESIAN_POINT ( 'NONE',  ( 150.0000000000000284, 15.00000000000000000, -49.99999999999998579 ) ) ;
#5448=EDGE_LOOP ( 'NONE', ( #1713, #3150, #2241, #4361 ) ) ;
#5449=DIRECTION ( 'NONE',  ( -1.000000000000000000, 0.000000000000000000, -0.000000000000000000 ) ) ;
#5457=( GEOMETRIC_REPRESENTATION_CONTEXT ( 3 ) GLOBAL_UNCERTAINTY_ASSIGNED_CONTEXT ( ( #4346 ) ) GLOBAL_UNIT_ASSIGNED_CONTEXT ( ( #3816, #4644, #5577 ) ) REPRESENTATION_CONTEXT ( 'NONE', 'WORKASPACE' ) );
#5474=ADVANCED_FACE ( 'NONE', ( #3423 ), #2970, .F. ) ;
#5484=CARTESIAN_POINT ( 'NONE',  ( 24.99999999999998224, 7.000000000000006217, -75.00000000000000000 ) ) ;
#5487=VECTOR ( 'NONE', #4026, 1000.000000000000000 ) ;
#5494=CARTESIAN_POINT ( 'NONE',  ( 137.4999999999999716, -7.000000000000011546, 75.00000000000000000 ) ) ;
#5495=DIRECTION ( 'NONE',  ( 0.000000000000000000, -1.000000000000000000, 0.000000000000000000 ) ) ;
#5496=DIRECTION ( 'NONE',  ( 0.000000000000000000, 0.000000000000000000, 1.000000000000000000 ) ) ;
#5500=DIRECTION ( 'NONE',  ( 1.000000000000000000, -0.000000000000000000, -0.000000000000000000 ) ) ;
#5503=ORIENTED_EDGE ( 'NONE', *, *, #1925, .T. ) ;
#5515=DIRECTION ( 'NONE',  ( 0.000000000000000000, -0.000000000000000000, -1.000000000000000000 ) ) ;
#5524=AXIS2_PLACEMENT_3D ( 'NONE', #2213, #3529, #3047 ) ;
#5525=ORIENTED_EDGE ( 'NONE', *, *, #677, .F. ) ;
#5528=VECTOR ( 'NONE', #339, 1000.000000000000000 ) ;
#5554=CYLINDRICAL_SURFACE ( 'NONE', #4162, 4.999999999999990230 ) ;
#5566=DIRECTION ( 'NONE',  ( 0.000000000000000000, 1.000000000000000000, 0.000000000000000000 ) ) ;
#5568=DIRECTION ( 'NONE',  ( 0.000000000000000000, 0.000000000000000000, 1.000000000000000000 ) ) ;
#5577=( NAMED_UNIT ( * ) SI_UNIT ( $, .STERADIAN. ) SOLID_ANGLE_UNIT ( ) );
#5584=CARTESIAN_POINT ( 'NONE',  ( 137.4999999999999716, 6.999999999999985789, 75.00000000000001421 ) ) ;
#5585=ORIENTED_EDGE ( 'NONE', *, *, #4323, .F. ) ;
#5587=ORIENTED_EDGE ( 'NONE', *, *, #4293, .F. ) ;
#5597=PLANE ( 'NONE',  #5714 ) ;
#5598=CARTESIAN_POINT ( 'NONE',  ( 24.99999999999998224, 7.000000000000006217, -75.00000000000000000 ) ) ;
#5603=DIRECTION ( 'NONE',  ( 0.000000000000000000, -1.000000000000000000, 0.000000000000000000 ) ) ;
#5619=LINE ( 'NONE', #3325, #1443 ) ;
#5623=CARTESIAN_POINT ( 'NONE',  ( 162.5000000000000000, 0.000000000000000000, -5.000000000000000000 ) ) ;
#5638=ORIENTED_EDGE ( 'NONE', *, *, #1490, .F. ) ;
#5643=EDGE_CURVE ( 'NONE', #1820, #3290, #814, .T. ) ;
#5648=ORIENTED_EDGE ( 'NONE', *, *, #3801, .F. ) ;
#5649=AXIS2_PLACEMENT_3D ( 'NONE', #964, #609, #5669 ) ;
#5656=DIRECTION ( 'NONE',  ( 0.000000000000000000, -0.000000000000000000, 1.000000000000000000 ) ) ;
#5667=ORIENTED_EDGE ( 'NONE', *, *, #5953, .T. ) ;
#5669=DIRECTION ( 'NONE',  ( 0.000000000000000000, 0.000000000000000000, -1.000000000000000000 ) ) ;
#5683=LINE ( 'NONE', #4389, #4947 ) ;
#5703=CARTESIAN_POINT ( 'NONE',  ( 162.4999999999999716, 6.999999999999985789, 65.00000000000000000 ) ) ;
#5714=AXIS2_PLACEMENT_3D ( 'NONE', #3777, #1441, #5496 ) ;
#5725=ORIENTED_EDGE ( 'NONE', *, *, #677, .T. ) ;
#5729=SURFACE_STYLE_USAGE ( .BOTH. , #1140 ) ;
#5756=CARTESIAN_POINT ( 'NONE',  ( 162.5000000000000000, 0.000000000000000000, 0.000000000000000000 ) ) ;
#5758=LINE ( 'NONE', #3518, #5346 ) ;
#5765=ADVANCED_FACE ( 'NONE', ( #3692 ), #2354, .F. ) ;
#5779=DIRECTION ( 'NONE',  ( 0.000000000000000000, -0.000000000000000000, -1.000000000000000000 ) ) ;
#5786=DIRECTION ( 'NONE',  ( 0.000000000000000000, 0.000000000000000000, -1.000000000000000000 ) ) ;
#5796=LINE ( 'NONE', #1243, #1815 ) ;
#5799=ORIENTED_EDGE ( 'NONE', *, *, #1751, .T. ) ;
#5800=ORIENTED_EDGE ( 'NONE', *, *, #4621, .T. ) ;
#5817=EDGE_LOOP ( 'NONE', ( #3919, #3255, #1798, #756 ) ) ;
#5819=AXIS2_PLACEMENT_3D ( 'NONE', #4944, #3570, #1781 ) ;
#5849=DIRECTION ( 'NONE',  ( 0.000000000000000000, 0.000000000000000000, 1.000000000000000000 ) ) ;
#5855=VERTEX_POINT ( 'NONE', #2336 ) ;
#5857=DIRECTION ( 'NONE',  ( 0.000000000000000000, 0.000000000000000000, -1.000000000000000000 ) ) ;
#5860=ORIENTED_EDGE ( 'NONE', *, *, #2976, .T. ) ;
#5862=DIRECTION ( 'NONE',  ( -0.000000000000000000, -1.000000000000000000, -0.000000000000000000 ) ) ;
#5881=VERTEX_POINT ( 'NONE', #1454 ) ;
#5882=SHAPE_REPRESENTATION ( 'movable block', ( #5080 ), #5457 ) ;
#5887=ORIENTED_EDGE ( 'NONE', *, *, #4432, .F. ) ;
#5891=CYLINDRICAL_SURFACE ( 'NONE', #1852, 4.999999999999990230 ) ;
#5898=LINE ( 'NONE', #1746, #5528 ) ;
#5906=AXIS2_PLACEMENT_3D ( 'NONE', #3931, #1692, #5786 ) ;
#5908=EDGE_CURVE ( 'NONE', #605, #3368, #3796, .T. ) ;
#5924=MECHANICAL_DESIGN_GEOMETRIC_PRESENTATION_REPRESENTATION('',(#2639),#989);
#5932=ORIENTED_EDGE ( 'NONE', *, *, #4293, .T. ) ;
#5935=CARTESIAN_POINT ( 'NONE',  ( 137.4999999999999716, 0.000000000000000000, -5.000000000000000000 ) ) ;
#5936=FACE_OUTER_BOUND ( 'NONE', #422, .T. ) ;
#5939=COLOUR_RGB ( '',0.8941176470588234615, 0.8941176470588234615, 0.8941176470588234615 ) ;
#5953=EDGE_CURVE ( 'NONE', #2345, #5415, #4714, .T. ) ;
#5993=COLOUR_RGB('Dark Blue',0.08,0.2,0.34);
#5994=FILL_AREA_STYLE_COLOUR('',#5993);
#5995=FILL_AREA_STYLE('',(#5994));
#5996=SURFACE_STYLE_FILL_AREA(#5995);
#5997=SURFACE_SIDE_STYLE('',(#5996));
#5998=SURFACE_STYLE_USAGE(.BOTH.,#5997);
#5999=PRESENTATION_STYLE_ASSIGNMENT((#5998));
ENDSEC;
END-ISO-10303-21;
